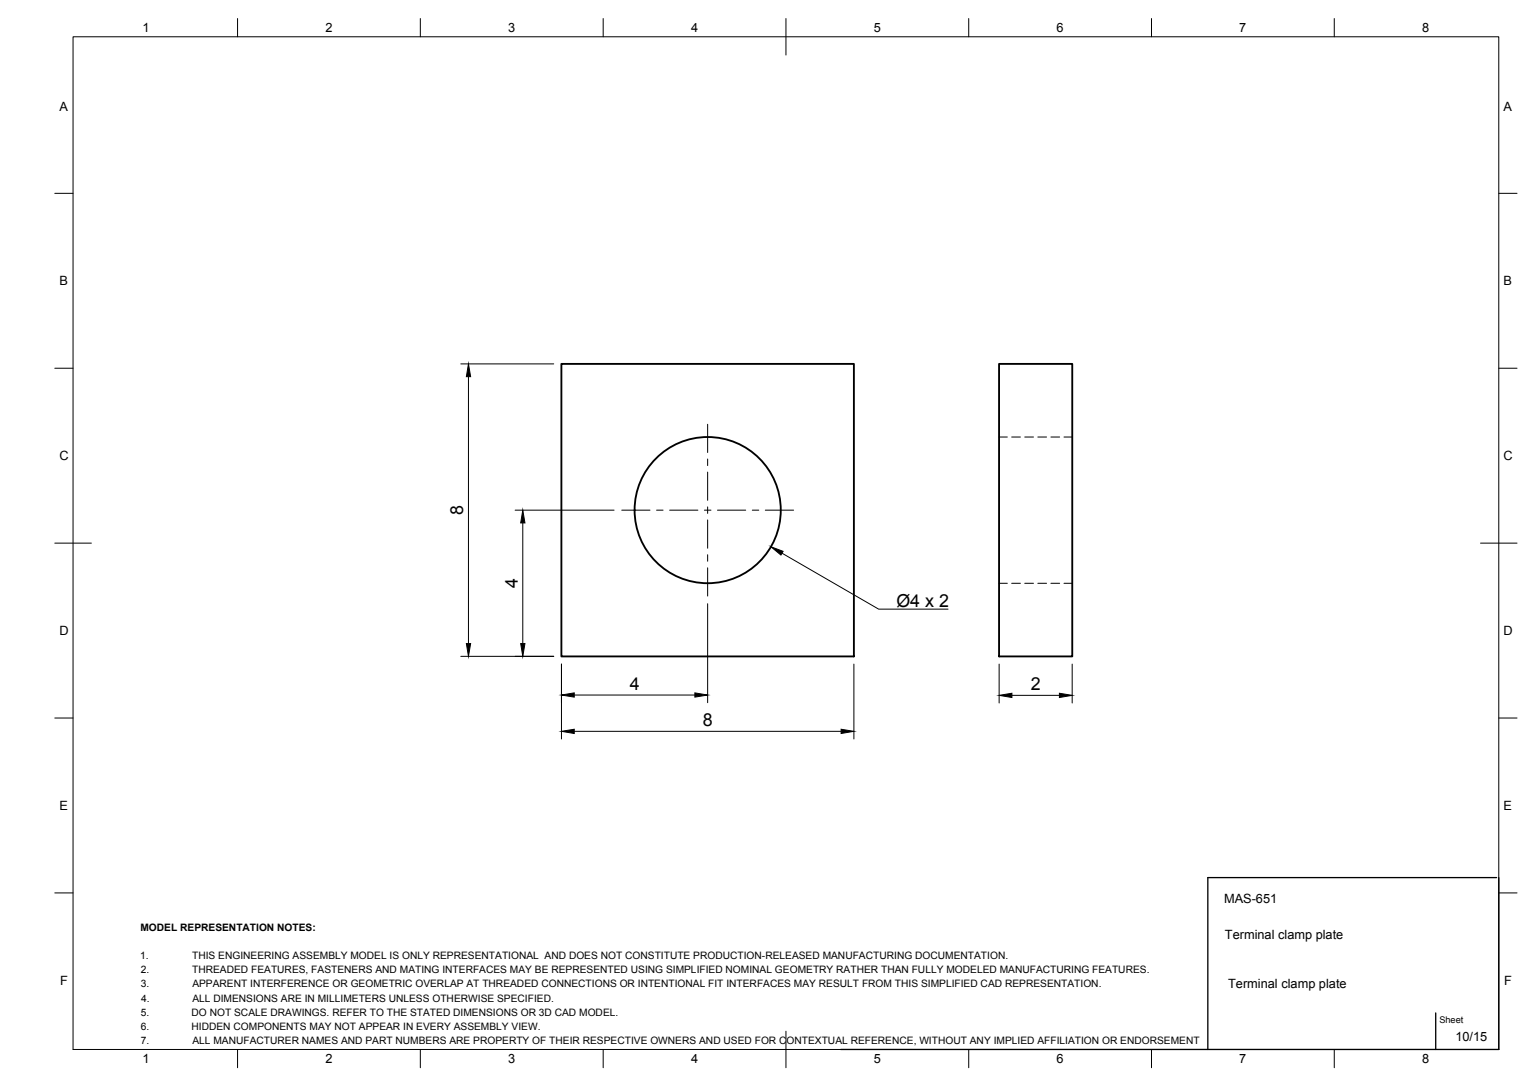
ISO-10303-21;
HEADER;
/* Generated by software containing ST-Developer
 * from STEP Tools, Inc. (www.steptools.com) 
 */

FILE_DESCRIPTION(
/* description */ ('Independent direct-acting normally-closed roller-plunger limit-switch
 CAD. Removable cover, insulated terminal supports, captured bus/conta
ct bridge, native Coil return spring, integral lower travel stop, reus
able instanced hardware and free roller. Manual geometric contact open
ing4mm; no snap-action/contact-force, electrical/current/voltage, envi
ronmental seal, safety-switch, wear, load or life certification. Exter
nal wiring and anchors omitted; fits and application engineering requi
red.'),
/* implementation_level */ '2;1');

FILE_NAME(
/* name */ 'Terminal clamp plate.step',
/* time_stamp */ '2026-11-08T07:32:43-08:00',
/* author */ (''),
/* organization */ (''),
/* preprocessor_version */ 'ST-DEVELOPER v20.2',
/* originating_system */ 'Autodesk Translation Framework v15.17.0.0',
/* authorisation */ '');

FILE_SCHEMA (('AUTOMOTIVE_DESIGN { 1 0 10303 214 3 1 1 }'));
ENDSEC;

DATA;
#10=MECHANICAL_DESIGN_GEOMETRIC_PRESENTATION_REPRESENTATION('',(#184),#36482);
#150=SHAPE_REPRESENTATION_RELATIONSHIP('SRR','None',#36563,#167);
#167=ADVANCED_BREP_SHAPE_REPRESENTATION('',(#201),#36473);
#184=STYLED_ITEM('',(#36656),#201);
#201=MANIFOLD_SOLID_BREP('Body1',#9775);
#287=FACE_BOUND('',#1404,.T.);
#288=FACE_BOUND('',#1406,.T.);
#388=PLANE('',#10447);
#389=PLANE('',#10448);
#390=PLANE('',#10449);
#391=PLANE('',#10450);
#392=PLANE('',#10451);
#393=PLANE('',#10452);
#808=FACE_OUTER_BOUND('',#1398,.T.);
#809=FACE_OUTER_BOUND('',#1399,.T.);
#810=FACE_OUTER_BOUND('',#1400,.T.);
#811=FACE_OUTER_BOUND('',#1401,.T.);
#812=FACE_OUTER_BOUND('',#1402,.T.);
#813=FACE_OUTER_BOUND('',#1403,.T.);
#814=FACE_OUTER_BOUND('',#1405,.T.);
#1398=EDGE_LOOP('',(#8008,#8009,#8010,#8011));
#1399=EDGE_LOOP('',(#8012,#8013,#8014,#8015));
#1400=EDGE_LOOP('',(#8016,#8017,#8018,#8019));
#1401=EDGE_LOOP('',(#8020,#8021,#8022,#8023));
#1402=EDGE_LOOP('',(#8024,#8025,#8026,#8027));
#1403=EDGE_LOOP('',(#8028,#8029,#8030,#8031));
#1404=EDGE_LOOP('',(#8032));
#1405=EDGE_LOOP('',(#8033,#8034,#8035,#8036));
#1406=EDGE_LOOP('',(#8037));
#1693=CIRCLE('',#10445,0.2);
#1694=CIRCLE('',#10446,0.2);
#2842=LINE('',#29214,#3416);
#2843=LINE('',#29219,#3417);
#2844=LINE('',#29221,#3418);
#2845=LINE('',#29223,#3419);
#2846=LINE('',#29224,#3420);
#2847=LINE('',#29227,#3421);
#2848=LINE('',#29229,#3422);
#2849=LINE('',#29230,#3423);
#2850=LINE('',#29233,#3424);
#2851=LINE('',#29235,#3425);
#2852=LINE('',#29236,#3426);
#2853=LINE('',#29238,#3427);
#2854=LINE('',#29239,#3428);
#3416=VECTOR('',#12035,0.2);
#3417=VECTOR('',#12040,1.);
#3418=VECTOR('',#12041,1.);
#3419=VECTOR('',#12042,1.);
#3420=VECTOR('',#12043,1.);
#3421=VECTOR('',#12046,1.);
#3422=VECTOR('',#12047,1.);
#3423=VECTOR('',#12048,1.);
#3424=VECTOR('',#12051,1.);
#3425=VECTOR('',#12052,1.);
#3426=VECTOR('',#12053,1.);
#3427=VECTOR('',#12056,1.);
#3428=VECTOR('',#12057,1.);
#4265=VERTEX_POINT('',#29211);
#4266=VERTEX_POINT('',#29213);
#4267=VERTEX_POINT('',#29217);
#4268=VERTEX_POINT('',#29218);
#4269=VERTEX_POINT('',#29220);
#4270=VERTEX_POINT('',#29222);
#4271=VERTEX_POINT('',#29226);
#4272=VERTEX_POINT('',#29228);
#4273=VERTEX_POINT('',#29232);
#4274=VERTEX_POINT('',#29234);
#5560=EDGE_CURVE('',#4265,#4265,#1693,.T.);
#5561=EDGE_CURVE('',#4265,#4266,#2842,.T.);
#5562=EDGE_CURVE('',#4266,#4266,#1694,.T.);
#5563=EDGE_CURVE('',#4267,#4268,#2843,.T.);
#5564=EDGE_CURVE('',#4268,#4269,#2844,.T.);
#5565=EDGE_CURVE('',#4270,#4269,#2845,.T.);
#5566=EDGE_CURVE('',#4267,#4270,#2846,.T.);
#5567=EDGE_CURVE('',#4271,#4267,#2847,.T.);
#5568=EDGE_CURVE('',#4272,#4270,#2848,.T.);
#5569=EDGE_CURVE('',#4271,#4272,#2849,.T.);
#5570=EDGE_CURVE('',#4273,#4271,#2850,.T.);
#5571=EDGE_CURVE('',#4274,#4272,#2851,.T.);
#5572=EDGE_CURVE('',#4273,#4274,#2852,.T.);
#5573=EDGE_CURVE('',#4268,#4273,#2853,.T.);
#5574=EDGE_CURVE('',#4269,#4274,#2854,.T.);
#8008=ORIENTED_EDGE('',*,*,#5560,.F.);
#8009=ORIENTED_EDGE('',*,*,#5561,.T.);
#8010=ORIENTED_EDGE('',*,*,#5562,.F.);
#8011=ORIENTED_EDGE('',*,*,#5561,.F.);
#8012=ORIENTED_EDGE('',*,*,#5563,.T.);
#8013=ORIENTED_EDGE('',*,*,#5564,.T.);
#8014=ORIENTED_EDGE('',*,*,#5565,.F.);
#8015=ORIENTED_EDGE('',*,*,#5566,.F.);
#8016=ORIENTED_EDGE('',*,*,#5567,.T.);
#8017=ORIENTED_EDGE('',*,*,#5566,.T.);
#8018=ORIENTED_EDGE('',*,*,#5568,.F.);
#8019=ORIENTED_EDGE('',*,*,#5569,.F.);
#8020=ORIENTED_EDGE('',*,*,#5570,.T.);
#8021=ORIENTED_EDGE('',*,*,#5569,.T.);
#8022=ORIENTED_EDGE('',*,*,#5571,.F.);
#8023=ORIENTED_EDGE('',*,*,#5572,.F.);
#8024=ORIENTED_EDGE('',*,*,#5573,.T.);
#8025=ORIENTED_EDGE('',*,*,#5572,.T.);
#8026=ORIENTED_EDGE('',*,*,#5574,.F.);
#8027=ORIENTED_EDGE('',*,*,#5564,.F.);
#8028=ORIENTED_EDGE('',*,*,#5574,.T.);
#8029=ORIENTED_EDGE('',*,*,#5571,.T.);
#8030=ORIENTED_EDGE('',*,*,#5568,.T.);
#8031=ORIENTED_EDGE('',*,*,#5565,.T.);
#8032=ORIENTED_EDGE('',*,*,#5560,.T.);
#8033=ORIENTED_EDGE('',*,*,#5573,.F.);
#8034=ORIENTED_EDGE('',*,*,#5563,.F.);
#8035=ORIENTED_EDGE('',*,*,#5567,.F.);
#8036=ORIENTED_EDGE('',*,*,#5570,.F.);
#8037=ORIENTED_EDGE('',*,*,#5562,.T.);
#9121=CYLINDRICAL_SURFACE('',#10444,0.2);
#9598=ADVANCED_FACE('',(#808),#9121,.F.);
#9599=ADVANCED_FACE('',(#809),#388,.T.);
#9600=ADVANCED_FACE('',(#810),#389,.T.);
#9601=ADVANCED_FACE('',(#811),#390,.T.);
#9602=ADVANCED_FACE('',(#812),#391,.T.);
#9603=ADVANCED_FACE('',(#813,#287),#392,.T.);
#9604=ADVANCED_FACE('',(#814,#288),#393,.F.);
#9775=CLOSED_SHELL('',(#9598,#9599,#9600,#9601,#9602,#9603,#9604));
#10443=AXIS2_PLACEMENT_3D('',#29209,#12029,#12030);
#10444=AXIS2_PLACEMENT_3D('',#29210,#12031,#12032);
#10445=AXIS2_PLACEMENT_3D('',#29212,#12033,#12034);
#10446=AXIS2_PLACEMENT_3D('',#29215,#12036,#12037);
#10447=AXIS2_PLACEMENT_3D('',#29216,#12038,#12039);
#10448=AXIS2_PLACEMENT_3D('',#29225,#12044,#12045);
#10449=AXIS2_PLACEMENT_3D('',#29231,#12049,#12050);
#10450=AXIS2_PLACEMENT_3D('',#29237,#12054,#12055);
#10451=AXIS2_PLACEMENT_3D('',#29240,#12058,#12059);
#10452=AXIS2_PLACEMENT_3D('',#29241,#12060,#12061);
#12029=DIRECTION('axis',(0.,0.,1.));
#12030=DIRECTION('refdir',(1.,0.,0.));
#12031=DIRECTION('center_axis',(0.,0.,-1.));
#12032=DIRECTION('ref_axis',(1.,0.,0.));
#12033=DIRECTION('center_axis',(0.,0.,-1.));
#12034=DIRECTION('ref_axis',(1.,0.,0.));
#12035=DIRECTION('',(0.,0.,-1.));
#12036=DIRECTION('center_axis',(0.,0.,1.));
#12037=DIRECTION('ref_axis',(1.,0.,0.));
#12038=DIRECTION('center_axis',(0.,1.,0.));
#12039=DIRECTION('ref_axis',(-1.,0.,0.));
#12040=DIRECTION('',(-1.,0.,0.));
#12041=DIRECTION('',(0.,0.,1.));
#12042=DIRECTION('',(-1.,0.,0.));
#12043=DIRECTION('',(0.,0.,1.));
#12044=DIRECTION('center_axis',(1.,0.,0.));
#12045=DIRECTION('ref_axis',(0.,1.,0.));
#12046=DIRECTION('',(0.,1.,0.));
#12047=DIRECTION('',(0.,1.,0.));
#12048=DIRECTION('',(0.,0.,1.));
#12049=DIRECTION('center_axis',(0.,-1.,0.));
#12050=DIRECTION('ref_axis',(1.,0.,0.));
#12051=DIRECTION('',(1.,0.,0.));
#12052=DIRECTION('',(1.,0.,0.));
#12053=DIRECTION('',(0.,0.,1.));
#12054=DIRECTION('center_axis',(-1.,0.,0.));
#12055=DIRECTION('ref_axis',(0.,-1.,0.));
#12056=DIRECTION('',(0.,-1.,0.));
#12057=DIRECTION('',(0.,-1.,0.));
#12058=DIRECTION('center_axis',(0.,0.,1.));
#12059=DIRECTION('ref_axis',(1.,0.,0.));
#12060=DIRECTION('center_axis',(0.,0.,1.));
#12061=DIRECTION('ref_axis',(1.,0.,0.));
#29209=CARTESIAN_POINT('',(0.,0.,0.));
#29210=CARTESIAN_POINT('Origin',(0.,0.,4.1));
#29211=CARTESIAN_POINT('',(-0.2,2.44929359829471E-17,4.2));
#29212=CARTESIAN_POINT('Origin',(0.,0.,4.2));
#29213=CARTESIAN_POINT('',(-0.2,2.44929359829471E-17,4.));
#29214=CARTESIAN_POINT('',(-0.2,2.44929359829471E-17,4.1));
#29215=CARTESIAN_POINT('Origin',(0.,0.,4.));
#29216=CARTESIAN_POINT('Origin',(0.4,0.4,4.));
#29217=CARTESIAN_POINT('',(0.4,0.4,4.));
#29218=CARTESIAN_POINT('',(-0.4,0.4,4.));
#29219=CARTESIAN_POINT('',(0.4,0.4,4.));
#29220=CARTESIAN_POINT('',(-0.4,0.4,4.2));
#29221=CARTESIAN_POINT('',(-0.4,0.4,4.));
#29222=CARTESIAN_POINT('',(0.4,0.4,4.2));
#29223=CARTESIAN_POINT('',(0.4,0.4,4.2));
#29224=CARTESIAN_POINT('',(0.4,0.4,4.));
#29225=CARTESIAN_POINT('Origin',(0.4,-0.4,4.));
#29226=CARTESIAN_POINT('',(0.4,-0.4,4.));
#29227=CARTESIAN_POINT('',(0.4,-0.4,4.));
#29228=CARTESIAN_POINT('',(0.4,-0.4,4.2));
#29229=CARTESIAN_POINT('',(0.4,-0.4,4.2));
#29230=CARTESIAN_POINT('',(0.4,-0.4,4.));
#29231=CARTESIAN_POINT('Origin',(-0.4,-0.4,4.));
#29232=CARTESIAN_POINT('',(-0.4,-0.4,4.));
#29233=CARTESIAN_POINT('',(-0.4,-0.4,4.));
#29234=CARTESIAN_POINT('',(-0.4,-0.4,4.2));
#29235=CARTESIAN_POINT('',(-0.4,-0.4,4.2));
#29236=CARTESIAN_POINT('',(-0.4,-0.4,4.));
#29237=CARTESIAN_POINT('Origin',(-0.4,0.4,4.));
#29238=CARTESIAN_POINT('',(-0.4,0.4,4.));
#29239=CARTESIAN_POINT('',(-0.4,0.4,4.2));
#29240=CARTESIAN_POINT('Origin',(0.,0.,4.2));
#29241=CARTESIAN_POINT('Origin',(0.,0.,4.));
#36454=UNCERTAINTY_MEASURE_WITH_UNIT(LENGTH_MEASURE(0.001),#36483,
'DISTANCE_ACCURACY_VALUE',
'Maximum model space distance between geometric entities at asserted c
onnectivities');
#36463=UNCERTAINTY_MEASURE_WITH_UNIT(LENGTH_MEASURE(0.001),#36483,
'DISTANCE_ACCURACY_VALUE',
'Maximum model space distance between geometric entities at asserted c
onnectivities');
#36473=(
GEOMETRIC_REPRESENTATION_CONTEXT(3)
GLOBAL_UNCERTAINTY_ASSIGNED_CONTEXT((#36454))
GLOBAL_UNIT_ASSIGNED_CONTEXT((#36483,#36485,#36486))
REPRESENTATION_CONTEXT('','3D')
);
#36482=(
GEOMETRIC_REPRESENTATION_CONTEXT(3)
GLOBAL_UNCERTAINTY_ASSIGNED_CONTEXT((#36463))
GLOBAL_UNIT_ASSIGNED_CONTEXT((#36483,#36485,#36486))
REPRESENTATION_CONTEXT('','3D')
);
#36483=(
LENGTH_UNIT()
NAMED_UNIT(*)
SI_UNIT(.CENTI.,.METRE.)
);
#36485=(
NAMED_UNIT(*)
PLANE_ANGLE_UNIT()
SI_UNIT($,.RADIAN.)
);
#36486=(
NAMED_UNIT(*)
SI_UNIT($,.STERADIAN.)
SOLID_ANGLE_UNIT()
);
#36496=SHAPE_DEFINITION_REPRESENTATION(#36514,#36563);
#36514=PRODUCT_DEFINITION_SHAPE('',$,#36582);
#36563=SHAPE_REPRESENTATION('',(#10443),#36473);
#36572=PRODUCT_DEFINITION_CONTEXT('part definition',#36628,'design');
#36582=PRODUCT_DEFINITION('Terminal clamp plate','Terminal clamp plate',
#36600,#36572);
#36600=PRODUCT_DEFINITION_FORMATION('',$,#36639);
#36628=APPLICATION_CONTEXT(
'Core Data for Automotive Mechanical Design Process');
#36629=PRODUCT_CONTEXT('part definition',#36628,'mechanical');
#36639=PRODUCT('Terminal clamp plate','Terminal clamp plate',$,(#36629));
#36656=PRESENTATION_STYLE_ASSIGNMENT((#36670));
#36670=SURFACE_STYLE_USAGE(.BOTH.,#36684);
#36684=SURFACE_SIDE_STYLE('',(#36698));
#36698=SURFACE_STYLE_FILL_AREA(#36712);
#36712=FILL_AREA_STYLE('Clamp gray',(#36726));
#36726=FILL_AREA_STYLE_COLOUR('Clamp gray',#36740);
#36740=COLOUR_RGB('Clamp gray',0.407843137254902,0.447058823529412,0.498039215686275);
ENDSEC;
END-ISO-10303-21;
